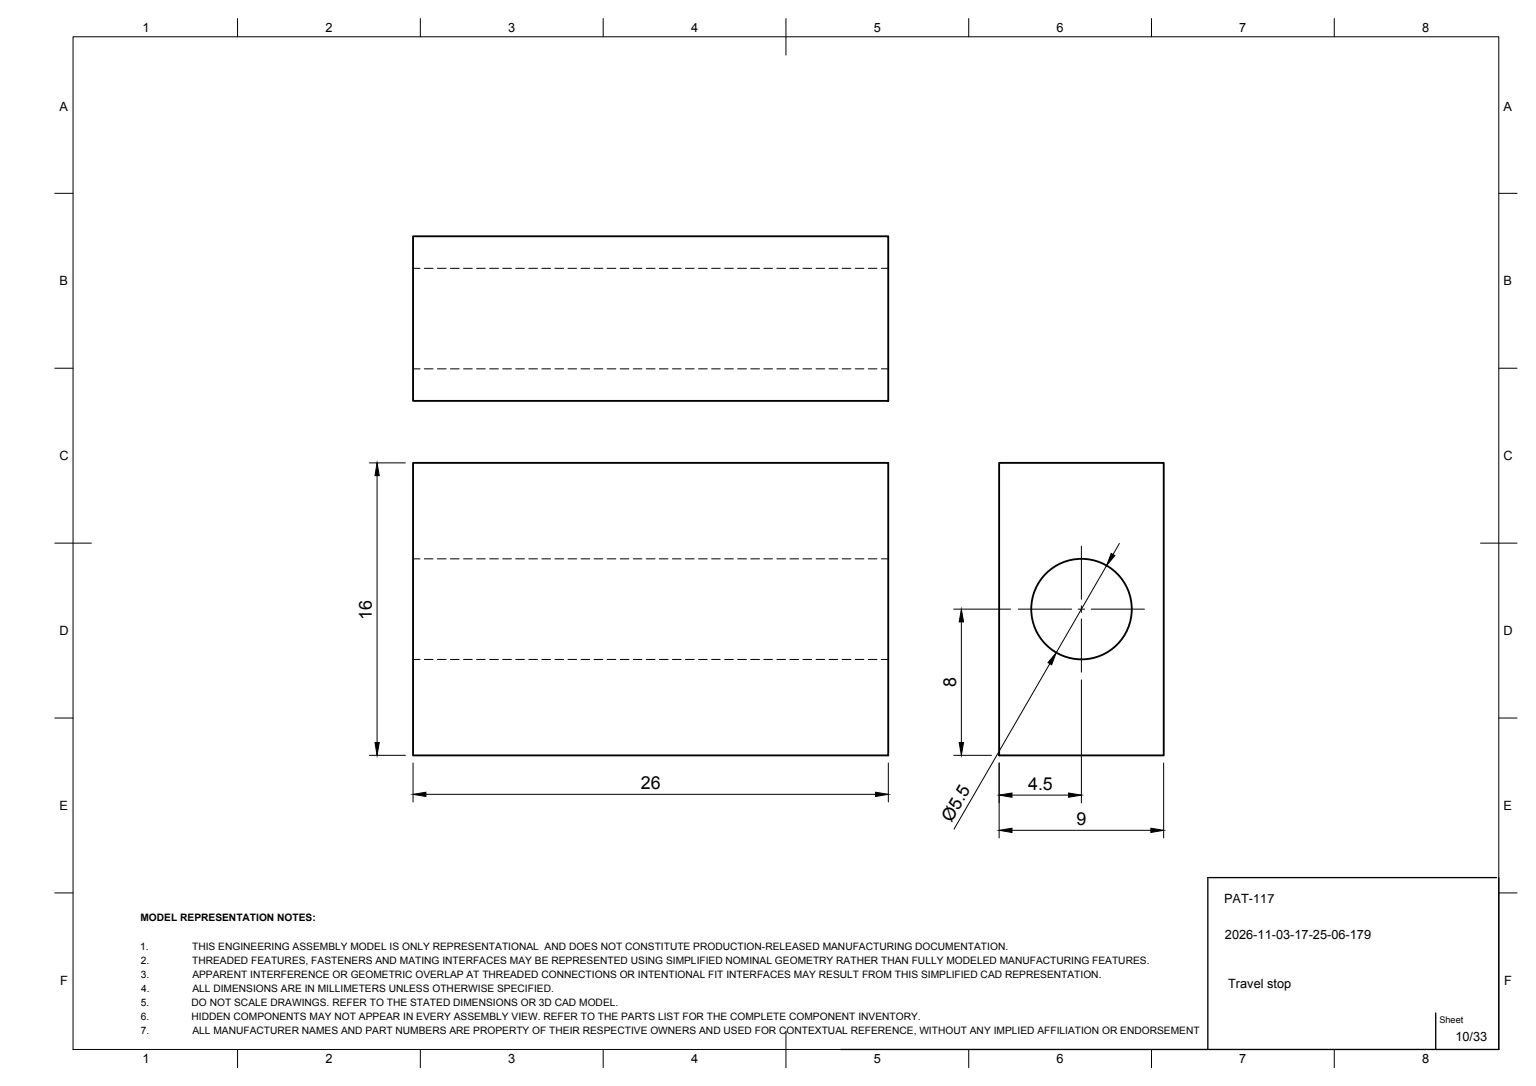
ISO-10303-21;
HEADER;
/* Generated by software containing ST-Developer
 * from STEP Tools, Inc. (www.steptools.com) 
 */

FILE_DESCRIPTION(
/* description */ ('Counterbalanced vertical column'),
/* implementation_level */ '2;1');

FILE_NAME(
/* name */ 'Travel stop.step',
/* time_stamp */ '2026-10-29T16:47:22-07:00',
/* author */ (''),
/* organization */ (''),
/* preprocessor_version */ 'ST-DEVELOPER v20.2',
/* originating_system */ 'Autodesk Translation Framework v15.17.0.0',
/* authorisation */ '');

FILE_SCHEMA (('AUTOMOTIVE_DESIGN { 1 0 10303 214 3 1 1 }'));
ENDSEC;

DATA;
#10=MECHANICAL_DESIGN_GEOMETRIC_PRESENTATION_REPRESENTATION('',(#355),#15040);
#285=SHAPE_REPRESENTATION_RELATIONSHIP('SRR','None',#15189,#320);
#320=ADVANCED_BREP_SHAPE_REPRESENTATION('',(#390),#15008);
#355=STYLED_ITEM('',(#15443),#390);
#390=MANIFOLD_SOLID_BREP('Body1',#7078);
#440=FACE_BOUND('',#1310,.T.);
#441=FACE_BOUND('',#1313,.T.);
#569=PLANE('',#7589);
#570=PLANE('',#7590);
#571=PLANE('',#7591);
#572=PLANE('',#7592);
#573=PLANE('',#7593);
#574=PLANE('',#7594);
#878=FACE_OUTER_BOUND('',#1307,.T.);
#879=FACE_OUTER_BOUND('',#1308,.T.);
#880=FACE_OUTER_BOUND('',#1309,.T.);
#881=FACE_OUTER_BOUND('',#1311,.T.);
#882=FACE_OUTER_BOUND('',#1312,.T.);
#883=FACE_OUTER_BOUND('',#1314,.T.);
#884=FACE_OUTER_BOUND('',#1315,.T.);
#1307=EDGE_LOOP('',(#5016,#5017,#5018,#5019));
#1308=EDGE_LOOP('',(#5020,#5021,#5022,#5023));
#1309=EDGE_LOOP('',(#5024,#5025,#5026,#5027));
#1310=EDGE_LOOP('',(#5028));
#1311=EDGE_LOOP('',(#5029,#5030,#5031,#5032));
#1312=EDGE_LOOP('',(#5033,#5034,#5035,#5036));
#1313=EDGE_LOOP('',(#5037));
#1314=EDGE_LOOP('',(#5038,#5039,#5040,#5041));
#1315=EDGE_LOOP('',(#5042,#5043,#5044,#5045));
#1837=LINE('',#10592,#2508);
#1838=LINE('',#10597,#2509);
#1839=LINE('',#10599,#2510);
#1840=LINE('',#10601,#2511);
#1841=LINE('',#10602,#2512);
#1842=LINE('',#10605,#2513);
#1843=LINE('',#10607,#2514);
#1844=LINE('',#10608,#2515);
#1845=LINE('',#10611,#2516);
#1846=LINE('',#10613,#2517);
#1847=LINE('',#10614,#2518);
#1848=LINE('',#10616,#2519);
#1849=LINE('',#10617,#2520);
#2508=VECTOR('',#8487,0.275);
#2509=VECTOR('',#8492,1.);
#2510=VECTOR('',#8493,1.);
#2511=VECTOR('',#8494,1.);
#2512=VECTOR('',#8495,1.);
#2513=VECTOR('',#8498,1.);
#2514=VECTOR('',#8499,1.);
#2515=VECTOR('',#8500,1.);
#2516=VECTOR('',#8503,1.);
#2517=VECTOR('',#8504,1.);
#2518=VECTOR('',#8505,1.);
#2519=VECTOR('',#8508,1.);
#2520=VECTOR('',#8509,1.);
#3121=CIRCLE('',#7587,0.275);
#3122=CIRCLE('',#7588,0.275);
#3382=VERTEX_POINT('',#10589);
#3383=VERTEX_POINT('',#10591);
#3384=VERTEX_POINT('',#10595);
#3385=VERTEX_POINT('',#10596);
#3386=VERTEX_POINT('',#10598);
#3387=VERTEX_POINT('',#10600);
#3388=VERTEX_POINT('',#10604);
#3389=VERTEX_POINT('',#10606);
#3390=VERTEX_POINT('',#10610);
#3391=VERTEX_POINT('',#10612);
#4009=EDGE_CURVE('',#3382,#3382,#3121,.T.);
#4010=EDGE_CURVE('',#3382,#3383,#1837,.T.);
#4011=EDGE_CURVE('',#3383,#3383,#3122,.T.);
#4012=EDGE_CURVE('',#3384,#3385,#1838,.T.);
#4013=EDGE_CURVE('',#3385,#3386,#1839,.T.);
#4014=EDGE_CURVE('',#3387,#3386,#1840,.T.);
#4015=EDGE_CURVE('',#3384,#3387,#1841,.T.);
#4016=EDGE_CURVE('',#3388,#3384,#1842,.T.);
#4017=EDGE_CURVE('',#3389,#3387,#1843,.T.);
#4018=EDGE_CURVE('',#3388,#3389,#1844,.T.);
#4019=EDGE_CURVE('',#3390,#3388,#1845,.T.);
#4020=EDGE_CURVE('',#3391,#3389,#1846,.T.);
#4021=EDGE_CURVE('',#3390,#3391,#1847,.T.);
#4022=EDGE_CURVE('',#3385,#3390,#1848,.T.);
#4023=EDGE_CURVE('',#3386,#3391,#1849,.T.);
#5016=ORIENTED_EDGE('',*,*,#4009,.F.);
#5017=ORIENTED_EDGE('',*,*,#4010,.T.);
#5018=ORIENTED_EDGE('',*,*,#4011,.F.);
#5019=ORIENTED_EDGE('',*,*,#4010,.F.);
#5020=ORIENTED_EDGE('',*,*,#4012,.T.);
#5021=ORIENTED_EDGE('',*,*,#4013,.T.);
#5022=ORIENTED_EDGE('',*,*,#4014,.F.);
#5023=ORIENTED_EDGE('',*,*,#4015,.F.);
#5024=ORIENTED_EDGE('',*,*,#4016,.T.);
#5025=ORIENTED_EDGE('',*,*,#4015,.T.);
#5026=ORIENTED_EDGE('',*,*,#4017,.F.);
#5027=ORIENTED_EDGE('',*,*,#4018,.F.);
#5028=ORIENTED_EDGE('',*,*,#4011,.T.);
#5029=ORIENTED_EDGE('',*,*,#4019,.T.);
#5030=ORIENTED_EDGE('',*,*,#4018,.T.);
#5031=ORIENTED_EDGE('',*,*,#4020,.F.);
#5032=ORIENTED_EDGE('',*,*,#4021,.F.);
#5033=ORIENTED_EDGE('',*,*,#4022,.T.);
#5034=ORIENTED_EDGE('',*,*,#4021,.T.);
#5035=ORIENTED_EDGE('',*,*,#4023,.F.);
#5036=ORIENTED_EDGE('',*,*,#4013,.F.);
#5037=ORIENTED_EDGE('',*,*,#4009,.T.);
#5038=ORIENTED_EDGE('',*,*,#4023,.T.);
#5039=ORIENTED_EDGE('',*,*,#4020,.T.);
#5040=ORIENTED_EDGE('',*,*,#4017,.T.);
#5041=ORIENTED_EDGE('',*,*,#4014,.T.);
#5042=ORIENTED_EDGE('',*,*,#4022,.F.);
#5043=ORIENTED_EDGE('',*,*,#4012,.F.);
#5044=ORIENTED_EDGE('',*,*,#4016,.F.);
#5045=ORIENTED_EDGE('',*,*,#4019,.F.);
#6588=CYLINDRICAL_SURFACE('',#7586,0.275);
#6720=ADVANCED_FACE('',(#878),#6588,.F.);
#6721=ADVANCED_FACE('',(#879),#569,.T.);
#6722=ADVANCED_FACE('',(#880,#440),#570,.T.);
#6723=ADVANCED_FACE('',(#881),#571,.T.);
#6724=ADVANCED_FACE('',(#882,#441),#572,.T.);
#6725=ADVANCED_FACE('',(#883),#573,.T.);
#6726=ADVANCED_FACE('',(#884),#574,.F.);
#7078=CLOSED_SHELL('',(#6720,#6721,#6722,#6723,#6724,#6725,#6726));
#7585=AXIS2_PLACEMENT_3D('',#10587,#8481,#8482);
#7586=AXIS2_PLACEMENT_3D('',#10588,#8483,#8484);
#7587=AXIS2_PLACEMENT_3D('',#10590,#8485,#8486);
#7588=AXIS2_PLACEMENT_3D('',#10593,#8488,#8489);
#7589=AXIS2_PLACEMENT_3D('',#10594,#8490,#8491);
#7590=AXIS2_PLACEMENT_3D('',#10603,#8496,#8497);
#7591=AXIS2_PLACEMENT_3D('',#10609,#8501,#8502);
#7592=AXIS2_PLACEMENT_3D('',#10615,#8506,#8507);
#7593=AXIS2_PLACEMENT_3D('',#10618,#8510,#8511);
#7594=AXIS2_PLACEMENT_3D('',#10619,#8512,#8513);
#8481=DIRECTION('axis',(0.,0.,1.));
#8482=DIRECTION('refdir',(1.,0.,0.));
#8483=DIRECTION('center_axis',(1.,0.,0.));
#8484=DIRECTION('ref_axis',(0.,0.,-1.));
#8485=DIRECTION('center_axis',(1.,0.,0.));
#8486=DIRECTION('ref_axis',(0.,0.,-1.));
#8487=DIRECTION('',(1.,0.,0.));
#8488=DIRECTION('center_axis',(-1.,0.,0.));
#8489=DIRECTION('ref_axis',(0.,0.,-1.));
#8490=DIRECTION('center_axis',(0.,1.,0.));
#8491=DIRECTION('ref_axis',(-1.,0.,0.));
#8492=DIRECTION('',(-1.,0.,0.));
#8493=DIRECTION('',(0.,0.,1.));
#8494=DIRECTION('',(-1.,0.,0.));
#8495=DIRECTION('',(0.,0.,1.));
#8496=DIRECTION('center_axis',(1.,0.,0.));
#8497=DIRECTION('ref_axis',(0.,1.,0.));
#8498=DIRECTION('',(0.,1.,0.));
#8499=DIRECTION('',(0.,1.,0.));
#8500=DIRECTION('',(0.,0.,1.));
#8501=DIRECTION('center_axis',(0.,-1.,0.));
#8502=DIRECTION('ref_axis',(1.,0.,0.));
#8503=DIRECTION('',(1.,0.,0.));
#8504=DIRECTION('',(1.,0.,0.));
#8505=DIRECTION('',(0.,0.,1.));
#8506=DIRECTION('center_axis',(-1.,0.,0.));
#8507=DIRECTION('ref_axis',(0.,-1.,0.));
#8508=DIRECTION('',(0.,-1.,0.));
#8509=DIRECTION('',(0.,-1.,0.));
#8510=DIRECTION('center_axis',(0.,0.,1.));
#8511=DIRECTION('ref_axis',(1.,0.,0.));
#8512=DIRECTION('center_axis',(0.,0.,1.));
#8513=DIRECTION('ref_axis',(1.,0.,0.));
#10587=CARTESIAN_POINT('',(0.,0.,0.));
#10588=CARTESIAN_POINT('Origin',(-1.5,2.,15.55));
#10589=CARTESIAN_POINT('',(-1.4,2.,15.825));
#10590=CARTESIAN_POINT('Origin',(-1.4,2.,15.55));
#10591=CARTESIAN_POINT('',(1.2,2.,15.825));
#10592=CARTESIAN_POINT('',(-1.5,2.,15.825));
#10593=CARTESIAN_POINT('Origin',(1.2,2.,15.55));
#10594=CARTESIAN_POINT('Origin',(1.2,2.8,15.1));
#10595=CARTESIAN_POINT('',(1.2,2.8,15.1));
#10596=CARTESIAN_POINT('',(-1.4,2.8,15.1));
#10597=CARTESIAN_POINT('',(1.2,2.8,15.1));
#10598=CARTESIAN_POINT('',(-1.4,2.8,16.));
#10599=CARTESIAN_POINT('',(-1.4,2.8,15.1));
#10600=CARTESIAN_POINT('',(1.2,2.8,16.));
#10601=CARTESIAN_POINT('',(1.2,2.8,16.));
#10602=CARTESIAN_POINT('',(1.2,2.8,15.1));
#10603=CARTESIAN_POINT('Origin',(1.2,1.2,15.1));
#10604=CARTESIAN_POINT('',(1.2,1.2,15.1));
#10605=CARTESIAN_POINT('',(1.2,1.2,15.1));
#10606=CARTESIAN_POINT('',(1.2,1.2,16.));
#10607=CARTESIAN_POINT('',(1.2,1.2,16.));
#10608=CARTESIAN_POINT('',(1.2,1.2,15.1));
#10609=CARTESIAN_POINT('Origin',(-1.4,1.2,15.1));
#10610=CARTESIAN_POINT('',(-1.4,1.2,15.1));
#10611=CARTESIAN_POINT('',(-1.4,1.2,15.1));
#10612=CARTESIAN_POINT('',(-1.4,1.2,16.));
#10613=CARTESIAN_POINT('',(-1.4,1.2,16.));
#10614=CARTESIAN_POINT('',(-1.4,1.2,15.1));
#10615=CARTESIAN_POINT('Origin',(-1.4,2.8,15.1));
#10616=CARTESIAN_POINT('',(-1.4,2.8,15.1));
#10617=CARTESIAN_POINT('',(-1.4,2.8,16.));
#10618=CARTESIAN_POINT('Origin',(-0.1,2.,16.));
#10619=CARTESIAN_POINT('Origin',(-0.1,2.,15.1));
#14968=UNCERTAINTY_MEASURE_WITH_UNIT(LENGTH_MEASURE(0.001),#15041,
'DISTANCE_ACCURACY_VALUE',
'Maximum model space distance between geometric entities at asserted c
onnectivities');
#15000=UNCERTAINTY_MEASURE_WITH_UNIT(LENGTH_MEASURE(0.001),#15041,
'DISTANCE_ACCURACY_VALUE',
'Maximum model space distance between geometric entities at asserted c
onnectivities');
#15008=(
GEOMETRIC_REPRESENTATION_CONTEXT(3)
GLOBAL_UNCERTAINTY_ASSIGNED_CONTEXT((#14968))
GLOBAL_UNIT_ASSIGNED_CONTEXT((#15041,#15043,#15044))
REPRESENTATION_CONTEXT('','3D')
);
#15040=(
GEOMETRIC_REPRESENTATION_CONTEXT(3)
GLOBAL_UNCERTAINTY_ASSIGNED_CONTEXT((#15000))
GLOBAL_UNIT_ASSIGNED_CONTEXT((#15041,#15043,#15044))
REPRESENTATION_CONTEXT('','3D')
);
#15041=(
LENGTH_UNIT()
NAMED_UNIT(*)
SI_UNIT(.CENTI.,.METRE.)
);
#15043=(
NAMED_UNIT(*)
PLANE_ANGLE_UNIT()
SI_UNIT($,.RADIAN.)
);
#15044=(
NAMED_UNIT(*)
SI_UNIT($,.STERADIAN.)
SOLID_ANGLE_UNIT()
);
#15052=SHAPE_DEFINITION_REPRESENTATION(#15091,#15189);
#15091=PRODUCT_DEFINITION_SHAPE('',$,#15229);
#15189=SHAPE_REPRESENTATION('',(#7585),#15008);
#15221=PRODUCT_DEFINITION_CONTEXT('part definition',#15340,'design');
#15229=PRODUCT_DEFINITION('Travel stop','Travel stop',#15268,#15221);
#15268=PRODUCT_DEFINITION_FORMATION('',$,#15349);
#15340=APPLICATION_CONTEXT(
'Core Data for Automotive Mechanical Design Process');
#15341=PRODUCT_CONTEXT('part definition',#15340,'mechanical');
#15349=PRODUCT('Travel stop','Travel stop','Travel stop',(#15341));
#15437=COLOUR_RGB('Light Blue',0.38,0.62,0.78);
#15438=FILL_AREA_STYLE_COLOUR('',#15437);
#15439=FILL_AREA_STYLE('',(#15438));
#15440=SURFACE_STYLE_FILL_AREA(#15439);
#15441=SURFACE_SIDE_STYLE('',(#15440));
#15442=SURFACE_STYLE_USAGE(.BOTH.,#15441);
#15443=PRESENTATION_STYLE_ASSIGNMENT((#15442));
ENDSEC;
END-ISO-10303-21;
